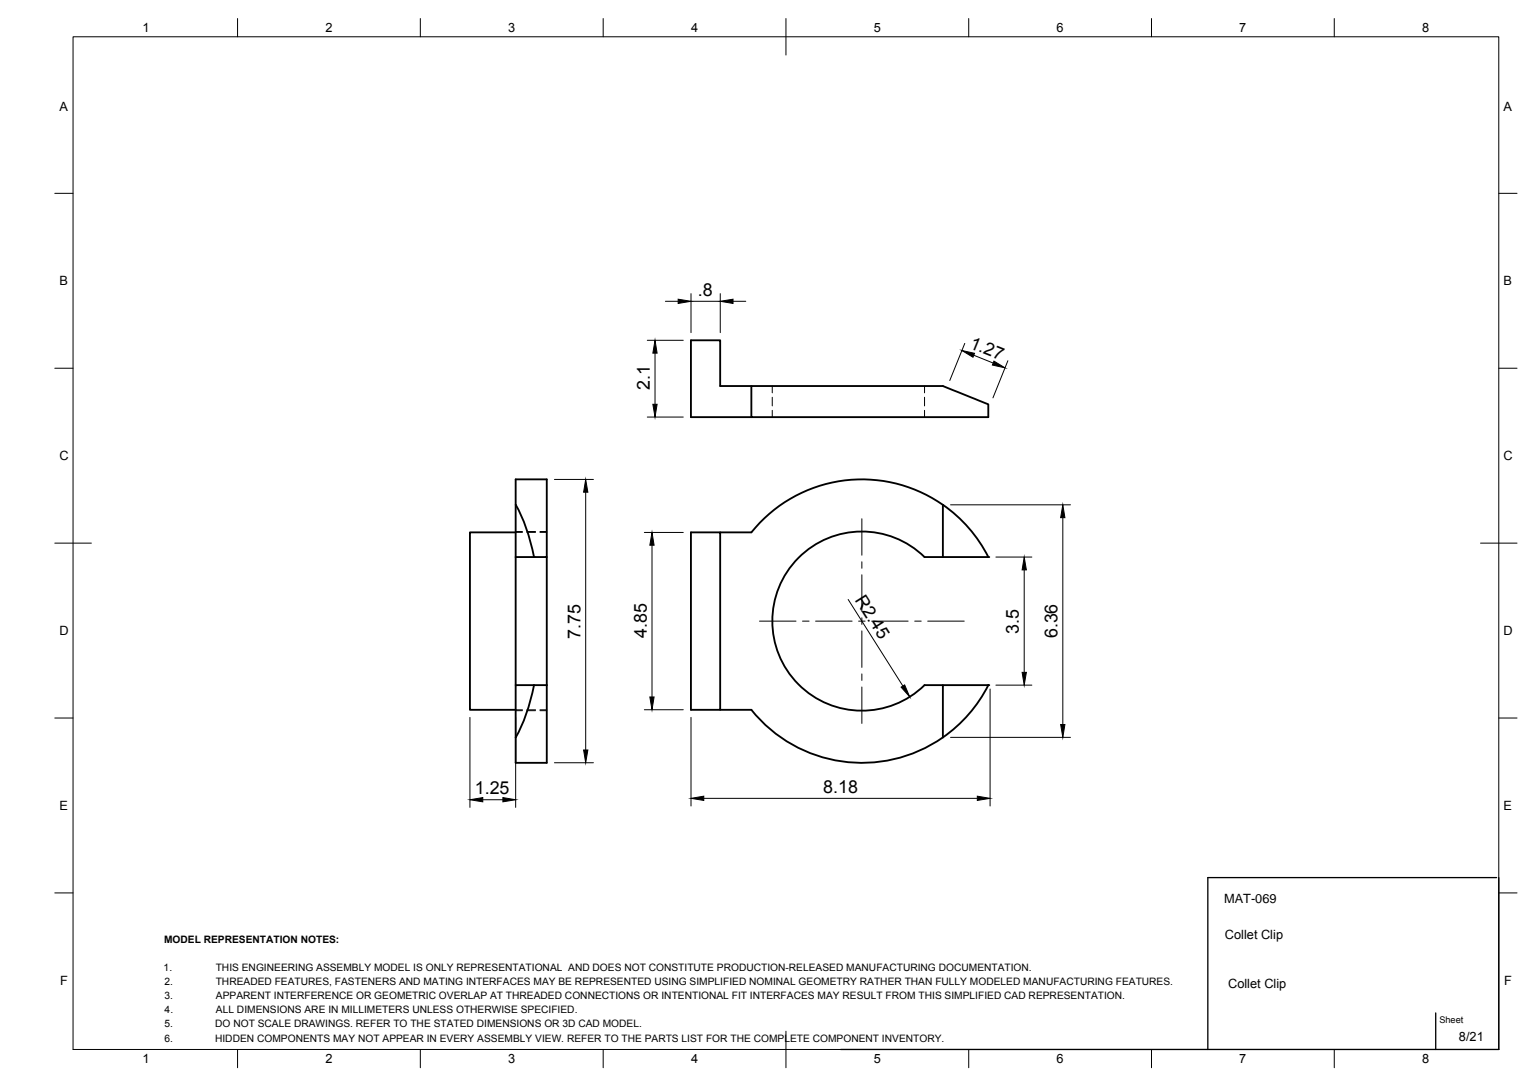
ISO-10303-21;
HEADER;
/* Generated by software containing ST-Developer
 * from STEP Tools, Inc. (www.steptools.com) 
 */

FILE_DESCRIPTION(
/* description */ ('CAx-IF Rec.Pracs.---Representation and Presentation of Product Manufa
cturing Information (PMI)---4.0---2014-10-13'),
/* implementation_level */ '2;1');

FILE_NAME(
/* name */ 'Collet Clip.step',
/* time_stamp */ '2026-10-24T15:08:39-07:00',
/* author */ (''),
/* organization */ (''),
/* preprocessor_version */ 'ST-DEVELOPER v20.2',
/* originating_system */ 'Autodesk Translation Framework v15.17.0.0',
/* authorisation */ '');

FILE_SCHEMA (('AP242_MANAGED_MODEL_BASED_3D_ENGINEERING_MIM_LF { 1 0 10303 442 2 1 4 }'));
ENDSEC;

DATA;
#10=MECHANICAL_DESIGN_GEOMETRIC_PRESENTATION_REPRESENTATION('',(#825),#50081);
#703=ELLIPSE('',#10402,0.00417722093727662,0.00387500000001);
#704=ELLIPSE('',#10406,0.00417722093727662,0.00387500000001);
#785=SHAPE_REPRESENTATION_RELATIONSHIP('SRR','None',#50153,#805);
#805=ADVANCED_BREP_SHAPE_REPRESENTATION('',(#845),#50066);
#825=STYLED_ITEM('',(#50259),#845);
#845=MANIFOLD_SOLID_BREP('Body1',#9870);
#941=PLANE('',#10401);
#942=PLANE('',#10403);
#943=PLANE('',#10405);
#944=PLANE('',#10407);
#945=PLANE('',#10412);
#946=PLANE('',#10413);
#947=PLANE('',#10414);
#948=PLANE('',#10415);
#949=PLANE('',#10416);
#950=PLANE('',#10423);
#951=PLANE('',#10424);
#952=PLANE('',#10425);
#953=PLANE('',#10426);
#1245=FACE_OUTER_BOUND('',#1817,.T.);
#1246=FACE_OUTER_BOUND('',#1818,.T.);
#1247=FACE_OUTER_BOUND('',#1819,.T.);
#1248=FACE_OUTER_BOUND('',#1820,.T.);
#1249=FACE_OUTER_BOUND('',#1821,.T.);
#1250=FACE_OUTER_BOUND('',#1822,.T.);
#1251=FACE_OUTER_BOUND('',#1823,.T.);
#1252=FACE_OUTER_BOUND('',#1824,.T.);
#1253=FACE_OUTER_BOUND('',#1825,.T.);
#1254=FACE_OUTER_BOUND('',#1826,.T.);
#1255=FACE_OUTER_BOUND('',#1827,.T.);
#1256=FACE_OUTER_BOUND('',#1828,.T.);
#1257=FACE_OUTER_BOUND('',#1829,.T.);
#1258=FACE_OUTER_BOUND('',#1830,.T.);
#1259=FACE_OUTER_BOUND('',#1831,.T.);
#1260=FACE_OUTER_BOUND('',#1832,.T.);
#1817=EDGE_LOOP('',(#6914,#6915,#6916,#6917));
#1818=EDGE_LOOP('',(#6918,#6919,#6920));
#1819=EDGE_LOOP('',(#6921,#6922,#6923,#6924));
#1820=EDGE_LOOP('',(#6925,#6926,#6927));
#1821=EDGE_LOOP('',(#6928,#6929,#6930,#6931,#6932,#6933));
#1822=EDGE_LOOP('',(#6934,#6935,#6936,#6937,#6938,#6939));
#1823=EDGE_LOOP('',(#6940,#6941,#6942,#6943,#6944,#6945));
#1824=EDGE_LOOP('',(#6946,#6947,#6948,#6949));
#1825=EDGE_LOOP('',(#6950,#6951,#6952,#6953));
#1826=EDGE_LOOP('',(#6954,#6955,#6956,#6957));
#1827=EDGE_LOOP('',(#6958,#6959,#6960,#6961));
#1828=EDGE_LOOP('',(#6962,#6963,#6964,#6965,#6966,#6967));
#1829=EDGE_LOOP('',(#6968,#6969,#6970,#6971,#6972,#6973));
#1830=EDGE_LOOP('',(#6974,#6975,#6976,#6977,#6978,#6979));
#1831=EDGE_LOOP('',(#6980,#6981,#6982,#6983,#6984,#6985,#6986,#6987,#6988,
#6989));
#1832=EDGE_LOOP('',(#6990,#6991,#6992,#6993,#6994,#6995,#6996,#6997));
#2365=LINE('',#17993,#2943);
#2366=LINE('',#17995,#2944);
#2367=LINE('',#17998,#2945);
#2368=LINE('',#18001,#2946);
#2369=LINE('',#18008,#2947);
#2370=LINE('',#18010,#2948);
#2371=LINE('',#18011,#2949);
#2372=LINE('',#18015,#2950);
#2373=LINE('',#18018,#2951);
#2374=LINE('',#18022,#2952);
#2375=LINE('',#18026,#2953);
#2376=LINE('',#18028,#2954);
#2377=LINE('',#18029,#2955);
#2378=LINE('',#18032,#2956);
#2379=LINE('',#18034,#2957);
#2380=LINE('',#18036,#2958);
#2381=LINE('',#18037,#2959);
#2382=LINE('',#18041,#2960);
#2383=LINE('',#18043,#2961);
#2384=LINE('',#18045,#2962);
#2385=LINE('',#18046,#2963);
#2386=LINE('',#18050,#2964);
#2387=LINE('',#18052,#2965);
#2388=LINE('',#18054,#2966);
#2389=LINE('',#18055,#2967);
#2390=LINE('',#18057,#2968);
#2391=LINE('',#18058,#2969);
#2392=LINE('',#18066,#2970);
#2393=LINE('',#18069,#2971);
#2394=LINE('',#18070,#2972);
#2395=LINE('',#18072,#2973);
#2396=LINE('',#18073,#2974);
#2943=VECTOR('',#11749,1.);
#2944=VECTOR('',#11750,1.);
#2945=VECTOR('',#11753,1.);
#2946=VECTOR('',#11756,1.);
#2947=VECTOR('',#11763,1.);
#2948=VECTOR('',#11764,1.);
#2949=VECTOR('',#11765,1.);
#2950=VECTOR('',#11770,1.);
#2951=VECTOR('',#11773,1.);
#2952=VECTOR('',#11776,1.);
#2953=VECTOR('',#11781,1.);
#2954=VECTOR('',#11782,1.);
#2955=VECTOR('',#11783,1.);
#2956=VECTOR('',#11786,1.);
#2957=VECTOR('',#11787,1.);
#2958=VECTOR('',#11788,1.);
#2959=VECTOR('',#11789,1.);
#2960=VECTOR('',#11792,1.);
#2961=VECTOR('',#11793,1.);
#2962=VECTOR('',#11794,1.);
#2963=VECTOR('',#11795,1.);
#2964=VECTOR('',#11798,1.);
#2965=VECTOR('',#11799,1.);
#2966=VECTOR('',#11800,1.);
#2967=VECTOR('',#11801,1.);
#2968=VECTOR('',#11804,1.);
#2969=VECTOR('',#11805,1.);
#2970=VECTOR('',#11816,1.);
#2971=VECTOR('',#11821,1.);
#2972=VECTOR('',#11822,1.);
#2973=VECTOR('',#11825,1.);
#2974=VECTOR('',#11826,1.);
#3530=CIRCLE('',#10404,0.00387500000001);
#3531=CIRCLE('',#10408,0.00387500000001);
#3532=CIRCLE('',#10410,0.00387500000001);
#3533=CIRCLE('',#10411,0.00387500000001);
#3534=CIRCLE('',#10418,0.00245000000001);
#3535=CIRCLE('',#10419,0.00245000000001);
#3536=CIRCLE('',#10421,0.00387500000001);
#3537=CIRCLE('',#10422,0.00387500000001);
#4010=VERTEX_POINT('',#17991);
#4011=VERTEX_POINT('',#17992);
#4012=VERTEX_POINT('',#17994);
#4013=VERTEX_POINT('',#17996);
#4014=VERTEX_POINT('',#18000);
#4015=VERTEX_POINT('',#18004);
#4016=VERTEX_POINT('',#18005);
#4017=VERTEX_POINT('',#18007);
#4018=VERTEX_POINT('',#18009);
#4019=VERTEX_POINT('',#18013);
#4020=VERTEX_POINT('',#18017);
#4021=VERTEX_POINT('',#18019);
#4022=VERTEX_POINT('',#18021);
#4023=VERTEX_POINT('',#18025);
#4024=VERTEX_POINT('',#18027);
#4025=VERTEX_POINT('',#18031);
#4026=VERTEX_POINT('',#18033);
#4027=VERTEX_POINT('',#18035);
#4028=VERTEX_POINT('',#18039);
#4029=VERTEX_POINT('',#18040);
#4030=VERTEX_POINT('',#18042);
#4031=VERTEX_POINT('',#18044);
#4032=VERTEX_POINT('',#18048);
#4033=VERTEX_POINT('',#18049);
#4034=VERTEX_POINT('',#18051);
#4035=VERTEX_POINT('',#18053);
#4036=VERTEX_POINT('',#18063);
#4037=VERTEX_POINT('',#18065);
#5110=EDGE_CURVE('',#4010,#4011,#2365,.T.);
#5111=EDGE_CURVE('',#4011,#4012,#2366,.T.);
#5112=EDGE_CURVE('',#4012,#4013,#703,.T.);
#5113=EDGE_CURVE('',#4010,#4013,#2367,.T.);
#5114=EDGE_CURVE('',#4014,#4011,#2368,.T.);
#5115=EDGE_CURVE('',#4012,#4014,#3530,.T.);
#5116=EDGE_CURVE('',#4015,#4016,#704,.T.);
#5117=EDGE_CURVE('',#4016,#4017,#2369,.T.);
#5118=EDGE_CURVE('',#4017,#4018,#2370,.T.);
#5119=EDGE_CURVE('',#4015,#4018,#2371,.T.);
#5120=EDGE_CURVE('',#4019,#4016,#3531,.T.);
#5121=EDGE_CURVE('',#4017,#4019,#2372,.T.);
#5122=EDGE_CURVE('',#4020,#4014,#2373,.T.);
#5123=EDGE_CURVE('',#4020,#4021,#3532,.T.);
#5124=EDGE_CURVE('',#4021,#4022,#2374,.T.);
#5125=EDGE_CURVE('',#4013,#4022,#3533,.T.);
#5126=EDGE_CURVE('',#4023,#4010,#2375,.T.);
#5127=EDGE_CURVE('',#4024,#4023,#2376,.T.);
#5128=EDGE_CURVE('',#4024,#4020,#2377,.T.);
#5129=EDGE_CURVE('',#4025,#4019,#2378,.T.);
#5130=EDGE_CURVE('',#4026,#4025,#2379,.T.);
#5131=EDGE_CURVE('',#4026,#4027,#2380,.T.);
#5132=EDGE_CURVE('',#4018,#4027,#2381,.T.);
#5133=EDGE_CURVE('',#4028,#4029,#2382,.T.);
#5134=EDGE_CURVE('',#4028,#4030,#2383,.T.);
#5135=EDGE_CURVE('',#4031,#4030,#2384,.T.);
#5136=EDGE_CURVE('',#4029,#4031,#2385,.T.);
#5137=EDGE_CURVE('',#4032,#4033,#2386,.T.);
#5138=EDGE_CURVE('',#4032,#4034,#2387,.T.);
#5139=EDGE_CURVE('',#4035,#4034,#2388,.T.);
#5140=EDGE_CURVE('',#4033,#4035,#2389,.T.);
#5141=EDGE_CURVE('',#4030,#4035,#2390,.T.);
#5142=EDGE_CURVE('',#4034,#4031,#2391,.T.);
#5143=EDGE_CURVE('',#4024,#4026,#3534,.T.);
#5144=EDGE_CURVE('',#4027,#4023,#3535,.T.);
#5145=EDGE_CURVE('',#4036,#4015,#3536,.T.);
#5146=EDGE_CURVE('',#4037,#4036,#2392,.T.);
#5147=EDGE_CURVE('',#4037,#4025,#3537,.T.);
#5148=EDGE_CURVE('',#4037,#4028,#2393,.T.);
#5149=EDGE_CURVE('',#4033,#4036,#2394,.T.);
#5150=EDGE_CURVE('',#4029,#4021,#2395,.T.);
#5151=EDGE_CURVE('',#4022,#4032,#2396,.T.);
#6914=ORIENTED_EDGE('',*,*,#5110,.T.);
#6915=ORIENTED_EDGE('',*,*,#5111,.T.);
#6916=ORIENTED_EDGE('',*,*,#5112,.T.);
#6917=ORIENTED_EDGE('',*,*,#5113,.F.);
#6918=ORIENTED_EDGE('',*,*,#5111,.F.);
#6919=ORIENTED_EDGE('',*,*,#5114,.F.);
#6920=ORIENTED_EDGE('',*,*,#5115,.F.);
#6921=ORIENTED_EDGE('',*,*,#5116,.T.);
#6922=ORIENTED_EDGE('',*,*,#5117,.T.);
#6923=ORIENTED_EDGE('',*,*,#5118,.T.);
#6924=ORIENTED_EDGE('',*,*,#5119,.F.);
#6925=ORIENTED_EDGE('',*,*,#5117,.F.);
#6926=ORIENTED_EDGE('',*,*,#5120,.F.);
#6927=ORIENTED_EDGE('',*,*,#5121,.F.);
#6928=ORIENTED_EDGE('',*,*,#5115,.T.);
#6929=ORIENTED_EDGE('',*,*,#5122,.F.);
#6930=ORIENTED_EDGE('',*,*,#5123,.T.);
#6931=ORIENTED_EDGE('',*,*,#5124,.T.);
#6932=ORIENTED_EDGE('',*,*,#5125,.F.);
#6933=ORIENTED_EDGE('',*,*,#5112,.F.);
#6934=ORIENTED_EDGE('',*,*,#5114,.T.);
#6935=ORIENTED_EDGE('',*,*,#5110,.F.);
#6936=ORIENTED_EDGE('',*,*,#5126,.F.);
#6937=ORIENTED_EDGE('',*,*,#5127,.F.);
#6938=ORIENTED_EDGE('',*,*,#5128,.T.);
#6939=ORIENTED_EDGE('',*,*,#5122,.T.);
#6940=ORIENTED_EDGE('',*,*,#5121,.T.);
#6941=ORIENTED_EDGE('',*,*,#5129,.F.);
#6942=ORIENTED_EDGE('',*,*,#5130,.F.);
#6943=ORIENTED_EDGE('',*,*,#5131,.T.);
#6944=ORIENTED_EDGE('',*,*,#5132,.F.);
#6945=ORIENTED_EDGE('',*,*,#5118,.F.);
#6946=ORIENTED_EDGE('',*,*,#5133,.F.);
#6947=ORIENTED_EDGE('',*,*,#5134,.T.);
#6948=ORIENTED_EDGE('',*,*,#5135,.F.);
#6949=ORIENTED_EDGE('',*,*,#5136,.F.);
#6950=ORIENTED_EDGE('',*,*,#5137,.F.);
#6951=ORIENTED_EDGE('',*,*,#5138,.T.);
#6952=ORIENTED_EDGE('',*,*,#5139,.F.);
#6953=ORIENTED_EDGE('',*,*,#5140,.F.);
#6954=ORIENTED_EDGE('',*,*,#5141,.T.);
#6955=ORIENTED_EDGE('',*,*,#5139,.T.);
#6956=ORIENTED_EDGE('',*,*,#5142,.T.);
#6957=ORIENTED_EDGE('',*,*,#5135,.T.);
#6958=ORIENTED_EDGE('',*,*,#5143,.F.);
#6959=ORIENTED_EDGE('',*,*,#5127,.T.);
#6960=ORIENTED_EDGE('',*,*,#5144,.F.);
#6961=ORIENTED_EDGE('',*,*,#5131,.F.);
#6962=ORIENTED_EDGE('',*,*,#5145,.F.);
#6963=ORIENTED_EDGE('',*,*,#5146,.F.);
#6964=ORIENTED_EDGE('',*,*,#5147,.T.);
#6965=ORIENTED_EDGE('',*,*,#5129,.T.);
#6966=ORIENTED_EDGE('',*,*,#5120,.T.);
#6967=ORIENTED_EDGE('',*,*,#5116,.F.);
#6968=ORIENTED_EDGE('',*,*,#5148,.F.);
#6969=ORIENTED_EDGE('',*,*,#5146,.T.);
#6970=ORIENTED_EDGE('',*,*,#5149,.F.);
#6971=ORIENTED_EDGE('',*,*,#5140,.T.);
#6972=ORIENTED_EDGE('',*,*,#5141,.F.);
#6973=ORIENTED_EDGE('',*,*,#5134,.F.);
#6974=ORIENTED_EDGE('',*,*,#5150,.F.);
#6975=ORIENTED_EDGE('',*,*,#5136,.T.);
#6976=ORIENTED_EDGE('',*,*,#5142,.F.);
#6977=ORIENTED_EDGE('',*,*,#5138,.F.);
#6978=ORIENTED_EDGE('',*,*,#5151,.F.);
#6979=ORIENTED_EDGE('',*,*,#5124,.F.);
#6980=ORIENTED_EDGE('',*,*,#5113,.T.);
#6981=ORIENTED_EDGE('',*,*,#5125,.T.);
#6982=ORIENTED_EDGE('',*,*,#5151,.T.);
#6983=ORIENTED_EDGE('',*,*,#5137,.T.);
#6984=ORIENTED_EDGE('',*,*,#5149,.T.);
#6985=ORIENTED_EDGE('',*,*,#5145,.T.);
#6986=ORIENTED_EDGE('',*,*,#5119,.T.);
#6987=ORIENTED_EDGE('',*,*,#5132,.T.);
#6988=ORIENTED_EDGE('',*,*,#5144,.T.);
#6989=ORIENTED_EDGE('',*,*,#5126,.T.);
#6990=ORIENTED_EDGE('',*,*,#5128,.F.);
#6991=ORIENTED_EDGE('',*,*,#5143,.T.);
#6992=ORIENTED_EDGE('',*,*,#5130,.T.);
#6993=ORIENTED_EDGE('',*,*,#5147,.F.);
#6994=ORIENTED_EDGE('',*,*,#5148,.T.);
#6995=ORIENTED_EDGE('',*,*,#5133,.T.);
#6996=ORIENTED_EDGE('',*,*,#5150,.T.);
#6997=ORIENTED_EDGE('',*,*,#5123,.F.);
#9177=CYLINDRICAL_SURFACE('',#10409,0.003875);
#9178=CYLINDRICAL_SURFACE('',#10417,0.00245);
#9179=CYLINDRICAL_SURFACE('',#10420,0.003875);
#9467=ADVANCED_FACE('',(#1245),#941,.T.);
#9468=ADVANCED_FACE('',(#1246),#942,.T.);
#9469=ADVANCED_FACE('',(#1247),#943,.T.);
#9470=ADVANCED_FACE('',(#1248),#944,.T.);
#9471=ADVANCED_FACE('',(#1249),#9177,.T.);
#9472=ADVANCED_FACE('',(#1250),#945,.T.);
#9473=ADVANCED_FACE('',(#1251),#946,.T.);
#9474=ADVANCED_FACE('',(#1252),#947,.T.);
#9475=ADVANCED_FACE('',(#1253),#948,.T.);
#9476=ADVANCED_FACE('',(#1254),#949,.T.);
#9477=ADVANCED_FACE('',(#1255),#9178,.F.);
#9478=ADVANCED_FACE('',(#1256),#9179,.T.);
#9479=ADVANCED_FACE('',(#1257),#950,.T.);
#9480=ADVANCED_FACE('',(#1258),#951,.T.);
#9481=ADVANCED_FACE('',(#1259),#952,.T.);
#9482=ADVANCED_FACE('',(#1260),#953,.F.);
#9870=CLOSED_SHELL('',(#9467,#9468,#9469,#9470,#9471,#9472,#9473,#9474,
#9475,#9476,#9477,#9478,#9479,#9480,#9481,#9482));
#10400=AXIS2_PLACEMENT_3D('',#17989,#11745,#11746);
#10401=AXIS2_PLACEMENT_3D('',#17990,#11747,#11748);
#10402=AXIS2_PLACEMENT_3D('',#17997,#11751,#11752);
#10403=AXIS2_PLACEMENT_3D('',#17999,#11754,#11755);
#10404=AXIS2_PLACEMENT_3D('',#18002,#11757,#11758);
#10405=AXIS2_PLACEMENT_3D('',#18003,#11759,#11760);
#10406=AXIS2_PLACEMENT_3D('',#18006,#11761,#11762);
#10407=AXIS2_PLACEMENT_3D('',#18012,#11766,#11767);
#10408=AXIS2_PLACEMENT_3D('',#18014,#11768,#11769);
#10409=AXIS2_PLACEMENT_3D('',#18016,#11771,#11772);
#10410=AXIS2_PLACEMENT_3D('',#18020,#11774,#11775);
#10411=AXIS2_PLACEMENT_3D('',#18023,#11777,#11778);
#10412=AXIS2_PLACEMENT_3D('',#18024,#11779,#11780);
#10413=AXIS2_PLACEMENT_3D('',#18030,#11784,#11785);
#10414=AXIS2_PLACEMENT_3D('',#18038,#11790,#11791);
#10415=AXIS2_PLACEMENT_3D('',#18047,#11796,#11797);
#10416=AXIS2_PLACEMENT_3D('',#18056,#11802,#11803);
#10417=AXIS2_PLACEMENT_3D('',#18059,#11806,#11807);
#10418=AXIS2_PLACEMENT_3D('',#18060,#11808,#11809);
#10419=AXIS2_PLACEMENT_3D('',#18061,#11810,#11811);
#10420=AXIS2_PLACEMENT_3D('',#18062,#11812,#11813);
#10421=AXIS2_PLACEMENT_3D('',#18064,#11814,#11815);
#10422=AXIS2_PLACEMENT_3D('',#18067,#11817,#11818);
#10423=AXIS2_PLACEMENT_3D('',#18068,#11819,#11820);
#10424=AXIS2_PLACEMENT_3D('',#18071,#11823,#11824);
#10425=AXIS2_PLACEMENT_3D('',#18074,#11827,#11828);
#10426=AXIS2_PLACEMENT_3D('',#18075,#11829,#11830);
#11745=DIRECTION('axis',(0.,0.,1.));
#11746=DIRECTION('refdir',(1.,0.,0.));
#11747=DIRECTION('center_axis',(0.,0.927650238806477,0.373450176653173));
#11748=DIRECTION('ref_axis',(-1.,0.,0.));
#11749=DIRECTION('',(0.,-0.373450176653687,0.92765023880627));
#11750=DIRECTION('',(1.,0.,0.));
#11751=DIRECTION('center_axis',(0.,0.927650238805982,0.373450176654402));
#11752=DIRECTION('ref_axis',(0.,0.373450176654402,-0.927650238805982));
#11753=DIRECTION('',(1.,0.,0.));
#11754=DIRECTION('center_axis',(0.,1.,1.09634523681734E-15));
#11755=DIRECTION('ref_axis',(1.,0.,0.));
#11756=DIRECTION('',(0.,1.09634523681734E-15,-1.));
#11757=DIRECTION('center_axis',(0.,-1.,-1.09634523681734E-15));
#11758=DIRECTION('ref_axis',(1.,0.,0.));
#11759=DIRECTION('center_axis',(0.,0.927650238806478,0.373450176653172));
#11760=DIRECTION('ref_axis',(-1.,0.,0.));
#11761=DIRECTION('center_axis',(0.,0.927650238805982,0.373450176654402));
#11762=DIRECTION('ref_axis',(0.,0.373450176654402,-0.927650238805982));
#11763=DIRECTION('',(1.,0.,0.));
#11764=DIRECTION('',(0.,0.373450176653686,-0.927650238806271));
#11765=DIRECTION('',(1.,0.,0.));
#11766=DIRECTION('center_axis',(0.,1.,1.09634523681734E-15));
#11767=DIRECTION('ref_axis',(1.,0.,0.));
#11768=DIRECTION('center_axis',(0.,-1.,-1.09634523681734E-15));
#11769=DIRECTION('ref_axis',(1.,0.,0.));
#11770=DIRECTION('',(0.,-1.09634523681734E-15,1.));
#11771=DIRECTION('center_axis',(0.,1.,1.09634523681734E-15));
#11772=DIRECTION('ref_axis',(1.,0.,0.));
#11773=DIRECTION('',(0.,1.,1.09634523681734E-15));
#11774=DIRECTION('center_axis',(0.,1.,1.09634523681734E-15));
#11775=DIRECTION('ref_axis',(1.,0.,0.));
#11776=DIRECTION('',(0.,1.,1.09634523681734E-15));
#11777=DIRECTION('center_axis',(0.,1.,1.09634523681734E-15));
#11778=DIRECTION('ref_axis',(1.,0.,0.));
#11779=DIRECTION('center_axis',(-1.,0.,0.));
#11780=DIRECTION('ref_axis',(0.,1.,1.09634523681734E-15));
#11781=DIRECTION('',(0.,-1.09634523681734E-15,1.));
#11782=DIRECTION('',(0.,1.,1.09634523681734E-15));
#11783=DIRECTION('',(0.,-1.09634523681734E-15,1.));
#11784=DIRECTION('center_axis',(1.,0.,0.));
#11785=DIRECTION('ref_axis',(0.,1.09634523681734E-15,-1.));
#11786=DIRECTION('',(0.,1.,1.09634523681734E-15));
#11787=DIRECTION('',(0.,-1.09634523681734E-15,1.));
#11788=DIRECTION('',(0.,1.,1.09634523681734E-15));
#11789=DIRECTION('',(0.,1.09634523681734E-15,-1.));
#11790=DIRECTION('center_axis',(0.,1.09634523681734E-15,-1.));
#11791=DIRECTION('ref_axis',(1.,0.,0.));
#11792=DIRECTION('',(1.,0.,0.));
#11793=DIRECTION('',(0.,1.,1.09634523681734E-15));
#11794=DIRECTION('',(-1.,0.,0.));
#11795=DIRECTION('',(0.,1.,1.09634523681734E-15));
#11796=DIRECTION('center_axis',(0.,-1.09634523681734E-15,1.));
#11797=DIRECTION('ref_axis',(0.,-1.,-1.09634523681734E-15));
#11798=DIRECTION('',(-1.,0.,0.));
#11799=DIRECTION('',(0.,1.,1.09634523681734E-15));
#11800=DIRECTION('',(1.,0.,0.));
#11801=DIRECTION('',(0.,1.,1.09634523681734E-15));
#11802=DIRECTION('center_axis',(0.,1.,1.09634523681734E-15));
#11803=DIRECTION('ref_axis',(1.,0.,0.));
#11804=DIRECTION('',(0.,-1.09634523681734E-15,1.));
#11805=DIRECTION('',(0.,1.09634523681734E-15,-1.));
#11806=DIRECTION('center_axis',(0.,1.,1.09634523681734E-15));
#11807=DIRECTION('ref_axis',(6.12323399573677E-17,1.09634523681734E-15,
-1.));
#11808=DIRECTION('center_axis',(0.,1.,1.09634523681734E-15));
#11809=DIRECTION('ref_axis',(1.,0.,0.));
#11810=DIRECTION('center_axis',(0.,-1.,-1.09634523681734E-15));
#11811=DIRECTION('ref_axis',(1.,0.,0.));
#11812=DIRECTION('center_axis',(0.,1.,1.09634523681734E-15));
#11813=DIRECTION('ref_axis',(-0.994617989425745,-1.13592451729936E-16,0.103610111044667));
#11814=DIRECTION('center_axis',(0.,1.,1.09634523681734E-15));
#11815=DIRECTION('ref_axis',(1.,0.,0.));
#11816=DIRECTION('',(0.,1.,1.09634523681734E-15));
#11817=DIRECTION('center_axis',(0.,1.,1.09634523681734E-15));
#11818=DIRECTION('ref_axis',(1.,0.,0.));
#11819=DIRECTION('center_axis',(-1.,0.,0.));
#11820=DIRECTION('ref_axis',(0.,1.,1.09634523681734E-15));
#11821=DIRECTION('',(0.,1.09634523681734E-15,-1.));
#11822=DIRECTION('',(0.,-1.09634523681734E-15,1.));
#11823=DIRECTION('center_axis',(1.,0.,0.));
#11824=DIRECTION('ref_axis',(0.,1.09634523681734E-15,-1.));
#11825=DIRECTION('',(0.,-1.09634523681734E-15,1.));
#11826=DIRECTION('',(0.,1.09634523681734E-15,-1.));
#11827=DIRECTION('center_axis',(0.,1.,1.09634523681734E-15));
#11828=DIRECTION('ref_axis',(1.,0.,0.));
#11829=DIRECTION('center_axis',(0.,1.,1.09634523681734E-15));
#11830=DIRECTION('ref_axis',(1.,0.,0.));
#17989=CARTESIAN_POINT('',(0.,0.,0.));
#17990=CARTESIAN_POINT('Origin',(0.00210744426613017,0.0161212256101277,
-0.00934021046660988));
#17991=CARTESIAN_POINT('',(0.00175,0.0163712256101277,-0.00996121046660988));
#17992=CARTESIAN_POINT('',(0.00175,0.0158712256101277,-0.00871921046660988));
#17993=CARTESIAN_POINT('',(0.00175000000001,0.0162735607568884,-0.00971861097112858));
#17994=CARTESIAN_POINT('',(0.00175135530812579,0.0158712256101277,-0.00871921046660988));
#17995=CARTESIAN_POINT('',(0.00210744426614017,0.0158712256101377,-0.00871921046659988));
#17996=CARTESIAN_POINT('',(0.00317977706452068,0.0163712256101277,-0.00996121046660988));
#17997=CARTESIAN_POINT('Origin',(0.,0.017262788742162,-0.0121758532865581));
#17998=CARTESIAN_POINT('',(0.00087500000001,0.0163712256101377,-0.00996121046659988));
#17999=CARTESIAN_POINT('Origin',(0.00246488853226034,0.0158712256101277,
-0.00933986729084157));
#18000=CARTESIAN_POINT('',(0.00175,0.0158712256101277,-0.00871852411507327));
#18001=CARTESIAN_POINT('',(0.00175000000001,0.0158712256101377,-0.00990053887871572));
#18002=CARTESIAN_POINT('Origin',(0.,0.0158712256101377,-0.0121758532865581));
#18003=CARTESIAN_POINT('Origin',(-0.00282233279839051,0.0161212256101277,
-0.00934021046660988));
#18004=CARTESIAN_POINT('',(-0.00317977706452068,0.0163712256101277,-0.00996121046660988));
#18005=CARTESIAN_POINT('',(-0.00175135530812579,0.0158712256101277,-0.00871921046660988));
#18006=CARTESIAN_POINT('Origin',(0.,0.017262788742162,-0.0121758532865581));
#18007=CARTESIAN_POINT('',(-0.00175,0.0158712256101277,-0.00871921046660988));
#18008=CARTESIAN_POINT('',(-0.00282233279840051,0.0158712256101377,-0.00871921046659988));
#18009=CARTESIAN_POINT('',(-0.00175,0.0163712256101277,-0.00996121046660988));
#18010=CARTESIAN_POINT('',(-0.00175000000001,0.0159717003423357,-0.00896878970137986));
#18011=CARTESIAN_POINT('',(-0.00158988853227034,0.0163712256101377,-0.00996121046659988));
#18012=CARTESIAN_POINT('Origin',(-0.00246488853226034,0.0158712256101277,
-0.00933986729084157));
#18013=CARTESIAN_POINT('',(-0.00175,0.0158712256101277,-0.00871852411507327));
#18014=CARTESIAN_POINT('Origin',(0.,0.0158712256101377,-0.0121758532865581));
#18015=CARTESIAN_POINT('',(-0.00175000000001,0.0158712256101377,-0.00902919570294742));
#18016=CARTESIAN_POINT('Origin',(0.,0.0155212256101277,-0.0121758532865581));
#18017=CARTESIAN_POINT('',(0.00175,0.0155212256101277,-0.00871852411507327));
#18018=CARTESIAN_POINT('',(0.00175000000001,0.0155212256101277,-0.00871852411506327));
#18019=CARTESIAN_POINT('',(0.002425,0.0155212256101277,-0.0151982695384996));
#18020=CARTESIAN_POINT('Origin',(0.,0.0155212256101277,-0.0121758532865581));
#18021=CARTESIAN_POINT('',(0.002425,0.0163712256101277,-0.0151982695384996));
#18022=CARTESIAN_POINT('',(0.00242500000001,0.0155212256101277,-0.0151982695385096));
#18023=CARTESIAN_POINT('Origin',(0.,0.0163712256101377,-0.0121758532865581));
#18024=CARTESIAN_POINT('Origin',(0.00175,0.0155212256101277,-0.0104612104666099));
#18025=CARTESIAN_POINT('',(0.00175,0.0163712256101277,-0.0104612104666099));
#18026=CARTESIAN_POINT('',(0.00175000000001,0.0163712256101377,-0.0121758532865581));
#18027=CARTESIAN_POINT('',(0.00175,0.0155212256101277,-0.0104612104666099));
#18028=CARTESIAN_POINT('',(0.00175000000001,0.0155212256101277,-0.0104612104665999));
#18029=CARTESIAN_POINT('',(0.00175000000001,0.0155212256101277,-0.0121758532865581));
#18030=CARTESIAN_POINT('Origin',(-0.00175,0.0155212256101277,-0.00871852411507327));
#18031=CARTESIAN_POINT('',(-0.00175,0.0155212256101277,-0.00871852411507327));
#18032=CARTESIAN_POINT('',(-0.00175000000001,0.0155212256101277,-0.00871852411506327));
#18033=CARTESIAN_POINT('',(-0.00175,0.0155212256101277,-0.0104612104666099));
#18034=CARTESIAN_POINT('',(-0.00175000000001,0.0155212256101277,-0.0121758532865581));
#18035=CARTESIAN_POINT('',(-0.00175,0.0163712256101277,-0.0104612104666099));
#18036=CARTESIAN_POINT('',(-0.00175000000001,0.0155212256101277,-0.0104612104665999));
#18037=CARTESIAN_POINT('',(-0.00175000000001,0.0163712256101377,-0.0121758532865581));
#18038=CARTESIAN_POINT('Origin',(0.002425,0.0155212256101277,-0.0168508532865581));
#18039=CARTESIAN_POINT('',(-0.002425,0.0155212256101277,-0.0168508532865581));
#18040=CARTESIAN_POINT('',(0.002425,0.0155212256101277,-0.0168508532865581));
#18041=CARTESIAN_POINT('',(-0.00242500000001,0.0155212256101277,-0.0168508532865681));
#18042=CARTESIAN_POINT('',(-0.002425,0.0176212256101277,-0.0168508532865581));
#18043=CARTESIAN_POINT('',(-0.00242500000001,0.0155212256101277,-0.0168508532865681));
#18044=CARTESIAN_POINT('',(0.002425,0.0176212256101277,-0.0168508532865581));
#18045=CARTESIAN_POINT('',(-0.00242500000001,0.0176212256101377,-0.0168508532865681));
#18046=CARTESIAN_POINT('',(0.00242500000001,0.0155212256101277,-0.0168508532865681));
#18047=CARTESIAN_POINT('Origin',(-0.002425,0.0155212256101277,-0.0160508532865581));
#18048=CARTESIAN_POINT('',(0.002425,0.0163712256101277,-0.0160508532865581));
#18049=CARTESIAN_POINT('',(-0.002425,0.0163712256101277,-0.0160508532865581));
#18050=CARTESIAN_POINT('',(-0.00242500000001,0.0163712256101377,-0.0160508532865681));
#18051=CARTESIAN_POINT('',(0.002425,0.0176212256101277,-0.0160508532865581));
#18052=CARTESIAN_POINT('',(0.00242500000001,0.0155212256101277,-0.0160508532865681));
#18053=CARTESIAN_POINT('',(-0.002425,0.0176212256101277,-0.0160508532865581));
#18054=CARTESIAN_POINT('',(-0.00242500000001,0.0176212256101377,-0.0160508532865681));
#18055=CARTESIAN_POINT('',(-0.00242500000001,0.0155212256101277,-0.0160508532865681));
#18056=CARTESIAN_POINT('Origin',(0.,0.0176212256101277,-0.0164508532865581));
#18057=CARTESIAN_POINT('',(-0.00242500000001,0.0176212256101377,-0.0160508532865681));
#18058=CARTESIAN_POINT('',(0.00242500000001,0.0176212256101377,-0.0168508532865681));
#18059=CARTESIAN_POINT('Origin',(0.,0.0155212256101277,-0.0121758532865581));
#18060=CARTESIAN_POINT('Origin',(0.,0.0155212256101277,-0.0121758532865581));
#18061=CARTESIAN_POINT('Origin',(0.,0.0163712256101377,-0.0121758532865581));
#18062=CARTESIAN_POINT('Origin',(0.,0.0155212256101277,-0.0121758532865581));
#18063=CARTESIAN_POINT('',(-0.002425,0.0163712256101277,-0.0151982695384996));
#18064=CARTESIAN_POINT('Origin',(0.,0.0163712256101377,-0.0121758532865581));
#18065=CARTESIAN_POINT('',(-0.002425,0.0155212256101277,-0.0151982695384996));
#18066=CARTESIAN_POINT('',(-0.00242500000001,0.0155212256101277,-0.0151982695385096));
#18067=CARTESIAN_POINT('Origin',(0.,0.0155212256101277,-0.0121758532865581));
#18068=CARTESIAN_POINT('Origin',(-0.002425,0.0155212256101277,-0.0160508532865581));
#18069=CARTESIAN_POINT('',(-0.00242500000001,0.0155212256101277,-0.0160508532865681));
#18070=CARTESIAN_POINT('',(-0.00242500000001,0.0163712256101377,-0.0151982695385096));
#18071=CARTESIAN_POINT('Origin',(0.002425,0.0155212256101277,-0.0151982695384996));
#18072=CARTESIAN_POINT('',(0.00242500000001,0.0155212256101277,-0.0160508532865681));
#18073=CARTESIAN_POINT('',(0.00242500000001,0.0163712256101377,-0.0160508532865681));
#18074=CARTESIAN_POINT('Origin',(0.,0.0163712256101277,-0.0123846887008157));
#18075=CARTESIAN_POINT('Origin',(0.,0.0155212256101277,-0.0123846887008157));
#50044=UNCERTAINTY_MEASURE_WITH_UNIT(LENGTH_MEASURE(1.E-5),#50082,
'DISTANCE_ACCURACY_VALUE',
'Maximum model space distance between geometric entities at asserted c
onnectivities');
#50059=UNCERTAINTY_MEASURE_WITH_UNIT(LENGTH_MEASURE(1.E-5),#50082,
'DISTANCE_ACCURACY_VALUE',
'Maximum model space distance between geometric entities at asserted c
onnectivities');
#50066=(
GEOMETRIC_REPRESENTATION_CONTEXT(3)
GLOBAL_UNCERTAINTY_ASSIGNED_CONTEXT((#50044))
GLOBAL_UNIT_ASSIGNED_CONTEXT((#50082,#50083,#50084))
REPRESENTATION_CONTEXT('','3D')
);
#50081=(
GEOMETRIC_REPRESENTATION_CONTEXT(3)
GLOBAL_UNCERTAINTY_ASSIGNED_CONTEXT((#50059))
GLOBAL_UNIT_ASSIGNED_CONTEXT((#50082,#50083,#50084))
REPRESENTATION_CONTEXT('','3D')
);
#50082=(
LENGTH_UNIT()
NAMED_UNIT(*)
SI_UNIT($,.METRE.)
);
#50083=(
NAMED_UNIT(*)
PLANE_ANGLE_UNIT()
SI_UNIT($,.RADIAN.)
);
#50084=(
NAMED_UNIT(*)
SI_UNIT($,.STERADIAN.)
SOLID_ANGLE_UNIT()
);
#50091=SHAPE_DEFINITION_REPRESENTATION(#50112,#50153);
#50112=PRODUCT_DEFINITION_SHAPE('',$,#50175);
#50153=SHAPE_REPRESENTATION('',(#10400),#50066);
#50168=PRODUCT_DEFINITION_CONTEXT('part definition',#50233,'design');
#50175=PRODUCT_DEFINITION('Collet Clip','Collet Clip',#50196,#50168);
#50196=PRODUCT_DEFINITION_FORMATION('',$,#50241);
#50233=APPLICATION_CONTEXT('Managed model based 3d engineering');
#50234=PRODUCT_CONTEXT('part definition',#50233,'mechanical');
#50241=PRODUCT('Collet Clip','Collet Clip',
'LEGAL AND USAGE DISCLAIMER: this Data/Model is provided \X2\201C\X0\A
S IS\X2\201D\X0\ for informational and representational only. It is a 
geometric approximation and is NOT engineered, certified, or guarantee
d for dimensional accuracy, exact tolerances, or production-level prec
ision. Vendor disclaims all implied warranties including fitness for a
 particular purpose. DO NOT USE FOR DIRECT PHYSICAL MANUFACTURING, AUT
OMATED PRODUCTION, OR SAFETY-CRITICAL SYSTEMS without independent engi
neering verification and resolution of any design discrepancies.',(#50234));
#50259=PRESENTATION_STYLE_ASSIGNMENT((#50266));
#50266=SURFACE_STYLE_USAGE(.BOTH.,#50273);
#50273=SURFACE_SIDE_STYLE('',(#50280));
#50280=SURFACE_STYLE_FILL_AREA(#50287);
#50287=FILL_AREA_STYLE('Opaque(246,246,243)',(#50294));
#50294=FILL_AREA_STYLE_COLOUR('Opaque(246,246,243)',#50301);
#50301=COLOUR_RGB('Opaque(246,246,243)',0.964705882352941,0.964705882352941,
0.952941176470588);
ENDSEC;
END-ISO-10303-21;
